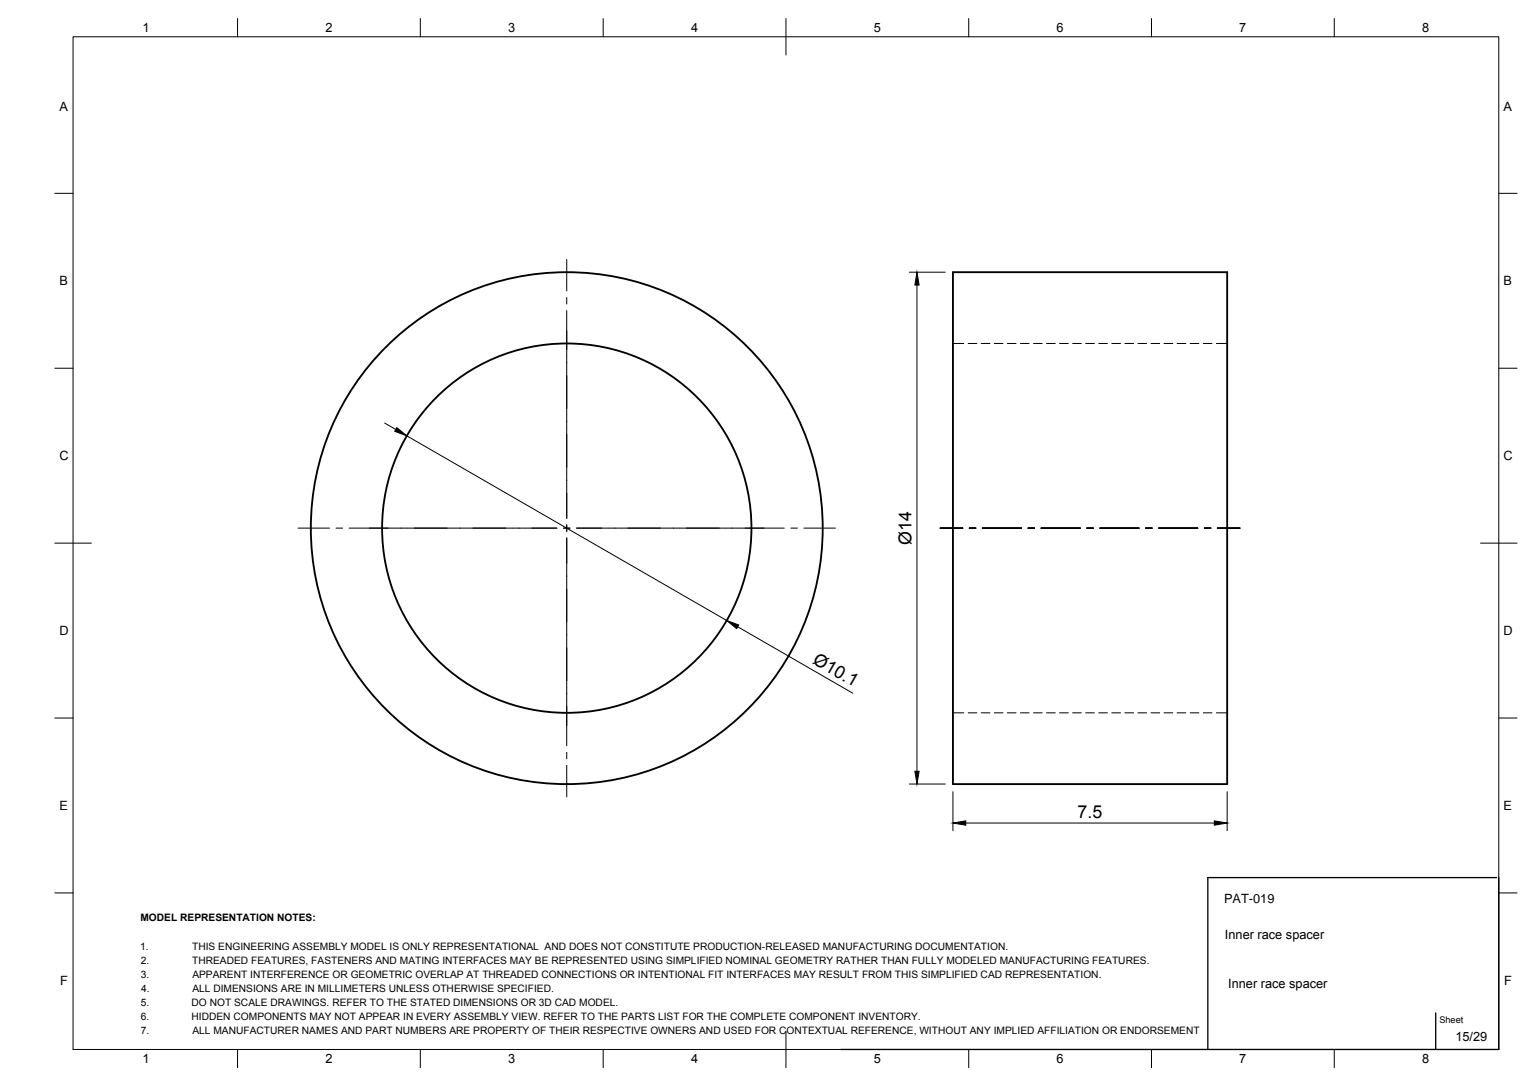
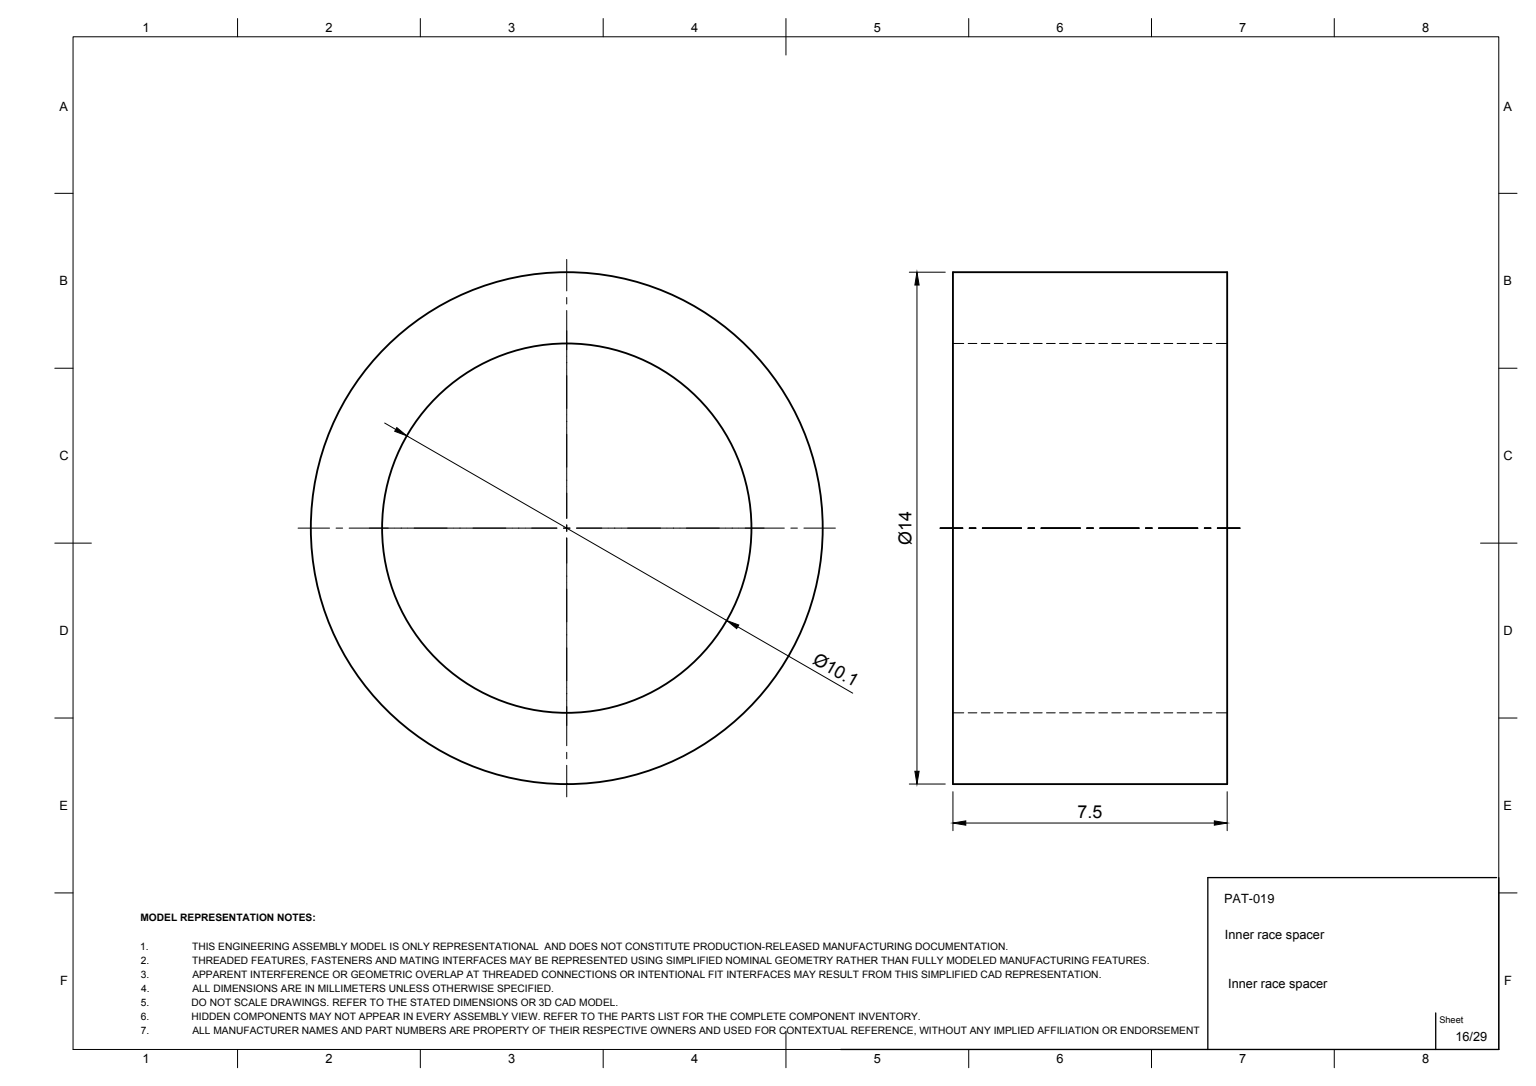
ISO-10303-21;
HEADER;
/* Generated by software containing ST-Developer
 * from STEP Tools, Inc. (www.steptools.com) 
 */

FILE_DESCRIPTION(
/* description */ ('Caster wheel assembly'),
/* implementation_level */ '2;1');

FILE_NAME(
/* name */ 'Inner race spacer.step',
/* time_stamp */ '2026-10-28T03:23:56-07:00',
/* author */ (''),
/* organization */ (''),
/* preprocessor_version */ 'ST-DEVELOPER v20.2',
/* originating_system */ 'Autodesk Translation Framework v15.17.0.0',
/* authorisation */ '');

FILE_SCHEMA (('AUTOMOTIVE_DESIGN { 1 0 10303 214 3 1 1 }'));
ENDSEC;

DATA;
#10=MECHANICAL_DESIGN_GEOMETRIC_PRESENTATION_REPRESENTATION('',(#232),#5385);
#188=SHAPE_REPRESENTATION_RELATIONSHIP('SRR','None',#5484,#210);
#210=ADVANCED_BREP_SHAPE_REPRESENTATION('',(#262),#5371);
#232=STYLED_ITEM('',(#5672),#262);
#262=MANIFOLD_SOLID_BREP('Body1',#2659);
#309=FACE_BOUND('',#693,.T.);
#310=FACE_BOUND('',#695,.T.);
#379=PLANE('',#3073);
#380=PLANE('',#3074);
#494=FACE_OUTER_BOUND('',#690,.T.);
#495=FACE_OUTER_BOUND('',#691,.T.);
#496=FACE_OUTER_BOUND('',#692,.T.);
#497=FACE_OUTER_BOUND('',#694,.T.);
#690=EDGE_LOOP('',(#2072,#2073,#2074,#2075));
#691=EDGE_LOOP('',(#2076,#2077,#2078,#2079));
#692=EDGE_LOOP('',(#2080));
#693=EDGE_LOOP('',(#2081));
#694=EDGE_LOOP('',(#2082));
#695=EDGE_LOOP('',(#2083));
#890=LINE('',#4561,#1024);
#891=LINE('',#4567,#1025);
#1024=VECTOR('',#3677,0.505);
#1025=VECTOR('',#3684,0.7);
#1129=CIRCLE('',#3068,0.505);
#1130=CIRCLE('',#3069,0.505);
#1131=CIRCLE('',#3071,0.7);
#1132=CIRCLE('',#3072,0.7);
#1332=VERTEX_POINT('',#4558);
#1333=VERTEX_POINT('',#4560);
#1334=VERTEX_POINT('',#4564);
#1335=VERTEX_POINT('',#4566);
#1604=EDGE_CURVE('',#1332,#1332,#1129,.T.);
#1605=EDGE_CURVE('',#1332,#1333,#890,.T.);
#1606=EDGE_CURVE('',#1333,#1333,#1130,.T.);
#1607=EDGE_CURVE('',#1334,#1334,#1131,.T.);
#1608=EDGE_CURVE('',#1334,#1335,#891,.T.);
#1609=EDGE_CURVE('',#1335,#1335,#1132,.T.);
#2072=ORIENTED_EDGE('',*,*,#1604,.F.);
#2073=ORIENTED_EDGE('',*,*,#1605,.T.);
#2074=ORIENTED_EDGE('',*,*,#1606,.T.);
#2075=ORIENTED_EDGE('',*,*,#1605,.F.);
#2076=ORIENTED_EDGE('',*,*,#1607,.F.);
#2077=ORIENTED_EDGE('',*,*,#1608,.T.);
#2078=ORIENTED_EDGE('',*,*,#1609,.T.);
#2079=ORIENTED_EDGE('',*,*,#1608,.F.);
#2080=ORIENTED_EDGE('',*,*,#1607,.T.);
#2081=ORIENTED_EDGE('',*,*,#1604,.T.);
#2082=ORIENTED_EDGE('',*,*,#1609,.F.);
#2083=ORIENTED_EDGE('',*,*,#1606,.F.);
#2453=CYLINDRICAL_SURFACE('',#3067,0.505);
#2454=CYLINDRICAL_SURFACE('',#3070,0.7);
#2554=ADVANCED_FACE('',(#494),#2453,.F.);
#2555=ADVANCED_FACE('',(#495),#2454,.T.);
#2556=ADVANCED_FACE('',(#496,#309),#379,.T.);
#2557=ADVANCED_FACE('',(#497,#310),#380,.F.);
#2659=CLOSED_SHELL('',(#2554,#2555,#2556,#2557));
#3066=AXIS2_PLACEMENT_3D('',#4556,#3671,#3672);
#3067=AXIS2_PLACEMENT_3D('',#4557,#3673,#3674);
#3068=AXIS2_PLACEMENT_3D('',#4559,#3675,#3676);
#3069=AXIS2_PLACEMENT_3D('',#4562,#3678,#3679);
#3070=AXIS2_PLACEMENT_3D('',#4563,#3680,#3681);
#3071=AXIS2_PLACEMENT_3D('',#4565,#3682,#3683);
#3072=AXIS2_PLACEMENT_3D('',#4568,#3685,#3686);
#3073=AXIS2_PLACEMENT_3D('',#4569,#3687,#3688);
#3074=AXIS2_PLACEMENT_3D('',#4570,#3689,#3690);
#3671=DIRECTION('axis',(0.,0.,1.));
#3672=DIRECTION('refdir',(1.,0.,0.));
#3673=DIRECTION('center_axis',(0.,1.,0.));
#3674=DIRECTION('ref_axis',(1.,0.,0.));
#3675=DIRECTION('center_axis',(0.,-1.,0.));
#3676=DIRECTION('ref_axis',(1.,0.,0.));
#3677=DIRECTION('',(0.,-1.,0.));
#3678=DIRECTION('center_axis',(0.,-1.,0.));
#3679=DIRECTION('ref_axis',(1.,0.,0.));
#3680=DIRECTION('center_axis',(0.,1.,0.));
#3681=DIRECTION('ref_axis',(1.,0.,0.));
#3682=DIRECTION('center_axis',(0.,1.,0.));
#3683=DIRECTION('ref_axis',(1.,0.,0.));
#3684=DIRECTION('',(0.,-1.,0.));
#3685=DIRECTION('center_axis',(0.,1.,0.));
#3686=DIRECTION('ref_axis',(1.,0.,0.));
#3687=DIRECTION('center_axis',(0.,1.,0.));
#3688=DIRECTION('ref_axis',(1.,0.,0.));
#3689=DIRECTION('center_axis',(0.,1.,0.));
#3690=DIRECTION('ref_axis',(1.,0.,0.));
#4556=CARTESIAN_POINT('',(0.,0.,0.));
#4557=CARTESIAN_POINT('Origin',(0.,-1.8,4.));
#4558=CARTESIAN_POINT('',(-0.505,-1.05,4.));
#4559=CARTESIAN_POINT('Origin',(0.,-1.05,4.));
#4560=CARTESIAN_POINT('',(-0.505,-1.8,4.));
#4561=CARTESIAN_POINT('',(-0.505,-1.8,4.));
#4562=CARTESIAN_POINT('Origin',(0.,-1.8,4.));
#4563=CARTESIAN_POINT('Origin',(0.,-1.8,4.));
#4564=CARTESIAN_POINT('',(-0.7,-1.05,4.));
#4565=CARTESIAN_POINT('Origin',(0.,-1.05,4.));
#4566=CARTESIAN_POINT('',(-0.7,-1.8,4.));
#4567=CARTESIAN_POINT('',(-0.7,-1.8,4.));
#4568=CARTESIAN_POINT('Origin',(0.,-1.8,4.));
#4569=CARTESIAN_POINT('Origin',(0.,-1.05,4.));
#4570=CARTESIAN_POINT('Origin',(0.,-1.8,4.));
#5343=UNCERTAINTY_MEASURE_WITH_UNIT(LENGTH_MEASURE(0.001),#5386,
'DISTANCE_ACCURACY_VALUE',
'Maximum model space distance between geometric entities at asserted c
onnectivities');
#5357=UNCERTAINTY_MEASURE_WITH_UNIT(LENGTH_MEASURE(0.001),#5386,
'DISTANCE_ACCURACY_VALUE',
'Maximum model space distance between geometric entities at asserted c
onnectivities');
#5371=(
GEOMETRIC_REPRESENTATION_CONTEXT(3)
GLOBAL_UNCERTAINTY_ASSIGNED_CONTEXT((#5343))
GLOBAL_UNIT_ASSIGNED_CONTEXT((#5386,#5388,#5389))
REPRESENTATION_CONTEXT('','3D')
);
#5385=(
GEOMETRIC_REPRESENTATION_CONTEXT(3)
GLOBAL_UNCERTAINTY_ASSIGNED_CONTEXT((#5357))
GLOBAL_UNIT_ASSIGNED_CONTEXT((#5386,#5388,#5389))
REPRESENTATION_CONTEXT('','3D')
);
#5386=(
LENGTH_UNIT()
NAMED_UNIT(*)
SI_UNIT(.CENTI.,.METRE.)
);
#5388=(
NAMED_UNIT(*)
PLANE_ANGLE_UNIT()
SI_UNIT($,.RADIAN.)
);
#5389=(
NAMED_UNIT(*)
SI_UNIT($,.STERADIAN.)
SOLID_ANGLE_UNIT()
);
#5403=SHAPE_DEFINITION_REPRESENTATION(#5435,#5484);
#5435=PRODUCT_DEFINITION_SHAPE('',$,#5512);
#5484=SHAPE_REPRESENTATION('',(#3066),#5371);
#5498=PRODUCT_DEFINITION_CONTEXT('part definition',#5581,'design');
#5512=PRODUCT_DEFINITION('Inner race spacer','Inner race spacer',#5539,
#5498);
#5539=PRODUCT_DEFINITION_FORMATION('',$,#5596);
#5581=APPLICATION_CONTEXT(
'Core Data for Automotive Mechanical Design Process');
#5582=PRODUCT_CONTEXT('part definition',#5581,'mechanical');
#5596=PRODUCT('Inner race spacer','Inner race spacer',
'Inner race spacer',(#5582));
#5666=COLOUR_RGB('Grey',0.48,0.52,0.57);
#5667=FILL_AREA_STYLE_COLOUR('',#5666);
#5668=FILL_AREA_STYLE('',(#5667));
#5669=SURFACE_STYLE_FILL_AREA(#5668);
#5670=SURFACE_SIDE_STYLE('',(#5669));
#5671=SURFACE_STYLE_USAGE(.BOTH.,#5670);
#5672=PRESENTATION_STYLE_ASSIGNMENT((#5671));
ENDSEC;
END-ISO-10303-21;
